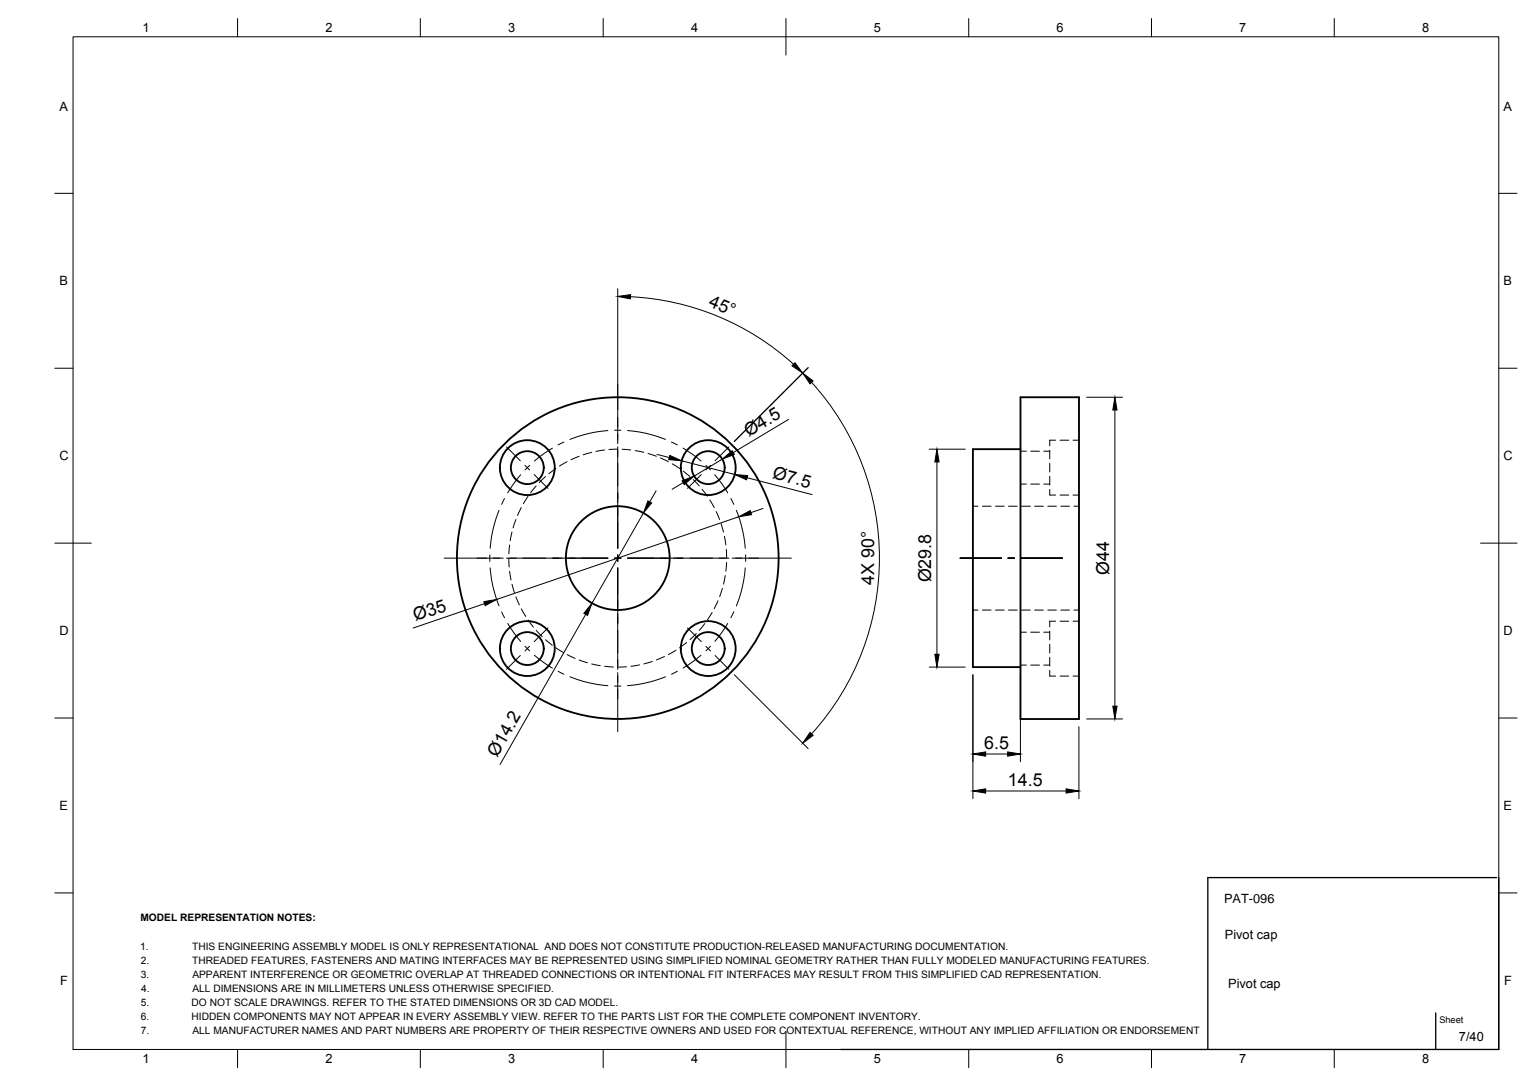
ISO-10303-21;
HEADER;
/* Generated by software containing ST-Developer
 * from STEP Tools, Inc. (www.steptools.com) 
 */

FILE_DESCRIPTION(
/* description */ ('PAT-096'),
/* implementation_level */ '2;1');

FILE_NAME(
/* name */ 'Pivot cap.step',
/* time_stamp */ '2026-10-29T17:03:14-07:00',
/* author */ (''),
/* organization */ (''),
/* preprocessor_version */ 'ST-DEVELOPER v20.2',
/* originating_system */ 'Autodesk Translation Framework v15.17.0.0',
/* authorisation */ '');

FILE_SCHEMA (('AUTOMOTIVE_DESIGN { 1 0 10303 214 3 1 1 }'));
ENDSEC;

DATA;
#10=MECHANICAL_DESIGN_GEOMETRIC_PRESENTATION_REPRESENTATION('',(#401),#10650);
#339=SHAPE_REPRESENTATION_RELATIONSHIP('SRR','None',#10799,#370);
#370=ADVANCED_BREP_SHAPE_REPRESENTATION('',(#439),#10617);
#401=STYLED_ITEM('',(#11050),#439);
#439=MANIFOLD_SOLID_BREP('Body1',#5535);
#508=FACE_BOUND('',#1222,.T.);
#509=FACE_BOUND('',#1225,.T.);
#510=FACE_BOUND('',#1228,.T.);
#511=FACE_BOUND('',#1231,.T.);
#512=FACE_BOUND('',#1238,.T.);
#513=FACE_BOUND('',#1242,.T.);
#514=FACE_BOUND('',#1243,.T.);
#515=FACE_BOUND('',#1244,.T.);
#516=FACE_BOUND('',#1245,.T.);
#517=FACE_BOUND('',#1246,.T.);
#518=FACE_BOUND('',#1248,.T.);
#519=FACE_BOUND('',#1249,.T.);
#520=FACE_BOUND('',#1250,.T.);
#521=FACE_BOUND('',#1251,.T.);
#522=FACE_BOUND('',#1252,.T.);
#641=PLANE('',#6046);
#642=PLANE('',#6051);
#643=PLANE('',#6056);
#644=PLANE('',#6061);
#645=PLANE('',#6074);
#646=PLANE('',#6081);
#647=PLANE('',#6082);
#849=FACE_OUTER_BOUND('',#1220,.T.);
#850=FACE_OUTER_BOUND('',#1221,.T.);
#851=FACE_OUTER_BOUND('',#1223,.T.);
#852=FACE_OUTER_BOUND('',#1224,.T.);
#853=FACE_OUTER_BOUND('',#1226,.T.);
#854=FACE_OUTER_BOUND('',#1227,.T.);
#855=FACE_OUTER_BOUND('',#1229,.T.);
#856=FACE_OUTER_BOUND('',#1230,.T.);
#857=FACE_OUTER_BOUND('',#1232,.T.);
#858=FACE_OUTER_BOUND('',#1233,.T.);
#859=FACE_OUTER_BOUND('',#1234,.T.);
#860=FACE_OUTER_BOUND('',#1235,.T.);
#861=FACE_OUTER_BOUND('',#1236,.T.);
#862=FACE_OUTER_BOUND('',#1237,.T.);
#863=FACE_OUTER_BOUND('',#1239,.T.);
#864=FACE_OUTER_BOUND('',#1240,.T.);
#865=FACE_OUTER_BOUND('',#1241,.T.);
#866=FACE_OUTER_BOUND('',#1247,.T.);
#1220=EDGE_LOOP('',(#3977,#3978,#3979,#3980));
#1221=EDGE_LOOP('',(#3981));
#1222=EDGE_LOOP('',(#3982));
#1223=EDGE_LOOP('',(#3983,#3984,#3985,#3986));
#1224=EDGE_LOOP('',(#3987));
#1225=EDGE_LOOP('',(#3988));
#1226=EDGE_LOOP('',(#3989,#3990,#3991,#3992));
#1227=EDGE_LOOP('',(#3993));
#1228=EDGE_LOOP('',(#3994));
#1229=EDGE_LOOP('',(#3995,#3996,#3997,#3998));
#1230=EDGE_LOOP('',(#3999));
#1231=EDGE_LOOP('',(#4000));
#1232=EDGE_LOOP('',(#4001,#4002,#4003,#4004));
#1233=EDGE_LOOP('',(#4005,#4006,#4007,#4008));
#1234=EDGE_LOOP('',(#4009,#4010,#4011,#4012));
#1235=EDGE_LOOP('',(#4013,#4014,#4015,#4016));
#1236=EDGE_LOOP('',(#4017,#4018,#4019,#4020));
#1237=EDGE_LOOP('',(#4021));
#1238=EDGE_LOOP('',(#4022));
#1239=EDGE_LOOP('',(#4023,#4024,#4025,#4026));
#1240=EDGE_LOOP('',(#4027,#4028,#4029,#4030));
#1241=EDGE_LOOP('',(#4031));
#1242=EDGE_LOOP('',(#4032));
#1243=EDGE_LOOP('',(#4033));
#1244=EDGE_LOOP('',(#4034));
#1245=EDGE_LOOP('',(#4035));
#1246=EDGE_LOOP('',(#4036));
#1247=EDGE_LOOP('',(#4037));
#1248=EDGE_LOOP('',(#4038));
#1249=EDGE_LOOP('',(#4039));
#1250=EDGE_LOOP('',(#4040));
#1251=EDGE_LOOP('',(#4041));
#1252=EDGE_LOOP('',(#4042));
#1665=LINE('',#8867,#1994);
#1666=LINE('',#8876,#1995);
#1667=LINE('',#8885,#1996);
#1668=LINE('',#8894,#1997);
#1669=LINE('',#8902,#1998);
#1670=LINE('',#8906,#1999);
#1671=LINE('',#8910,#2000);
#1672=LINE('',#8914,#2001);
#1673=LINE('',#8919,#2002);
#1674=LINE('',#8927,#2003);
#1675=LINE('',#8932,#2004);
#1994=VECTOR('',#6995,0.375);
#1995=VECTOR('',#7006,0.375);
#1996=VECTOR('',#7017,0.375);
#1997=VECTOR('',#7028,0.375);
#1998=VECTOR('',#7039,0.225);
#1999=VECTOR('',#7044,0.225);
#2000=VECTOR('',#7049,0.225);
#2001=VECTOR('',#7054,0.225);
#2002=VECTOR('',#7059,1.49);
#2003=VECTOR('',#7070,0.71);
#2004=VECTOR('',#7075,2.2);
#2322=CIRCLE('',#6044,0.375);
#2323=CIRCLE('',#6045,0.375);
#2324=CIRCLE('',#6047,0.225);
#2325=CIRCLE('',#6049,0.375);
#2326=CIRCLE('',#6050,0.375);
#2327=CIRCLE('',#6052,0.225);
#2328=CIRCLE('',#6054,0.375);
#2329=CIRCLE('',#6055,0.375);
#2330=CIRCLE('',#6057,0.225);
#2331=CIRCLE('',#6059,0.375);
#2332=CIRCLE('',#6060,0.375);
#2333=CIRCLE('',#6062,0.225);
#2334=CIRCLE('',#6064,0.225);
#2335=CIRCLE('',#6066,0.225);
#2336=CIRCLE('',#6068,0.225);
#2337=CIRCLE('',#6070,0.225);
#2338=CIRCLE('',#6072,1.49);
#2339=CIRCLE('',#6073,1.49);
#2340=CIRCLE('',#6075,0.71);
#2341=CIRCLE('',#6077,0.71);
#2342=CIRCLE('',#6079,2.2);
#2343=CIRCLE('',#6080,2.2);
#2665=VERTEX_POINT('',#8864);
#2666=VERTEX_POINT('',#8866);
#2667=VERTEX_POINT('',#8870);
#2668=VERTEX_POINT('',#8873);
#2669=VERTEX_POINT('',#8875);
#2670=VERTEX_POINT('',#8879);
#2671=VERTEX_POINT('',#8882);
#2672=VERTEX_POINT('',#8884);
#2673=VERTEX_POINT('',#8888);
#2674=VERTEX_POINT('',#8891);
#2675=VERTEX_POINT('',#8893);
#2676=VERTEX_POINT('',#8897);
#2677=VERTEX_POINT('',#8900);
#2678=VERTEX_POINT('',#8904);
#2679=VERTEX_POINT('',#8908);
#2680=VERTEX_POINT('',#8912);
#2681=VERTEX_POINT('',#8916);
#2682=VERTEX_POINT('',#8918);
#2683=VERTEX_POINT('',#8922);
#2684=VERTEX_POINT('',#8925);
#2685=VERTEX_POINT('',#8929);
#2686=VERTEX_POINT('',#8931);
#3167=EDGE_CURVE('',#2665,#2665,#2322,.T.);
#3168=EDGE_CURVE('',#2665,#2666,#1665,.T.);
#3169=EDGE_CURVE('',#2666,#2666,#2323,.T.);
#3170=EDGE_CURVE('',#2667,#2667,#2324,.T.);
#3171=EDGE_CURVE('',#2668,#2668,#2325,.T.);
#3172=EDGE_CURVE('',#2668,#2669,#1666,.T.);
#3173=EDGE_CURVE('',#2669,#2669,#2326,.T.);
#3174=EDGE_CURVE('',#2670,#2670,#2327,.T.);
#3175=EDGE_CURVE('',#2671,#2671,#2328,.T.);
#3176=EDGE_CURVE('',#2671,#2672,#1667,.T.);
#3177=EDGE_CURVE('',#2672,#2672,#2329,.T.);
#3178=EDGE_CURVE('',#2673,#2673,#2330,.T.);
#3179=EDGE_CURVE('',#2674,#2674,#2331,.T.);
#3180=EDGE_CURVE('',#2674,#2675,#1668,.T.);
#3181=EDGE_CURVE('',#2675,#2675,#2332,.T.);
#3182=EDGE_CURVE('',#2676,#2676,#2333,.T.);
#3183=EDGE_CURVE('',#2677,#2677,#2334,.T.);
#3184=EDGE_CURVE('',#2677,#2667,#1669,.T.);
#3185=EDGE_CURVE('',#2678,#2678,#2335,.T.);
#3186=EDGE_CURVE('',#2678,#2670,#1670,.T.);
#3187=EDGE_CURVE('',#2679,#2679,#2336,.T.);
#3188=EDGE_CURVE('',#2679,#2673,#1671,.T.);
#3189=EDGE_CURVE('',#2680,#2680,#2337,.T.);
#3190=EDGE_CURVE('',#2680,#2676,#1672,.T.);
#3191=EDGE_CURVE('',#2681,#2681,#2338,.T.);
#3192=EDGE_CURVE('',#2681,#2682,#1673,.T.);
#3193=EDGE_CURVE('',#2682,#2682,#2339,.T.);
#3194=EDGE_CURVE('',#2683,#2683,#2340,.T.);
#3195=EDGE_CURVE('',#2684,#2684,#2341,.T.);
#3196=EDGE_CURVE('',#2684,#2683,#1674,.T.);
#3197=EDGE_CURVE('',#2685,#2685,#2342,.T.);
#3198=EDGE_CURVE('',#2685,#2686,#1675,.T.);
#3199=EDGE_CURVE('',#2686,#2686,#2343,.T.);
#3977=ORIENTED_EDGE('',*,*,#3167,.F.);
#3978=ORIENTED_EDGE('',*,*,#3168,.T.);
#3979=ORIENTED_EDGE('',*,*,#3169,.F.);
#3980=ORIENTED_EDGE('',*,*,#3168,.F.);
#3981=ORIENTED_EDGE('',*,*,#3167,.T.);
#3982=ORIENTED_EDGE('',*,*,#3170,.F.);
#3983=ORIENTED_EDGE('',*,*,#3171,.F.);
#3984=ORIENTED_EDGE('',*,*,#3172,.T.);
#3985=ORIENTED_EDGE('',*,*,#3173,.F.);
#3986=ORIENTED_EDGE('',*,*,#3172,.F.);
#3987=ORIENTED_EDGE('',*,*,#3171,.T.);
#3988=ORIENTED_EDGE('',*,*,#3174,.F.);
#3989=ORIENTED_EDGE('',*,*,#3175,.F.);
#3990=ORIENTED_EDGE('',*,*,#3176,.T.);
#3991=ORIENTED_EDGE('',*,*,#3177,.F.);
#3992=ORIENTED_EDGE('',*,*,#3176,.F.);
#3993=ORIENTED_EDGE('',*,*,#3175,.T.);
#3994=ORIENTED_EDGE('',*,*,#3178,.F.);
#3995=ORIENTED_EDGE('',*,*,#3179,.F.);
#3996=ORIENTED_EDGE('',*,*,#3180,.T.);
#3997=ORIENTED_EDGE('',*,*,#3181,.F.);
#3998=ORIENTED_EDGE('',*,*,#3180,.F.);
#3999=ORIENTED_EDGE('',*,*,#3179,.T.);
#4000=ORIENTED_EDGE('',*,*,#3182,.F.);
#4001=ORIENTED_EDGE('',*,*,#3183,.F.);
#4002=ORIENTED_EDGE('',*,*,#3184,.T.);
#4003=ORIENTED_EDGE('',*,*,#3170,.T.);
#4004=ORIENTED_EDGE('',*,*,#3184,.F.);
#4005=ORIENTED_EDGE('',*,*,#3185,.F.);
#4006=ORIENTED_EDGE('',*,*,#3186,.T.);
#4007=ORIENTED_EDGE('',*,*,#3174,.T.);
#4008=ORIENTED_EDGE('',*,*,#3186,.F.);
#4009=ORIENTED_EDGE('',*,*,#3187,.F.);
#4010=ORIENTED_EDGE('',*,*,#3188,.T.);
#4011=ORIENTED_EDGE('',*,*,#3178,.T.);
#4012=ORIENTED_EDGE('',*,*,#3188,.F.);
#4013=ORIENTED_EDGE('',*,*,#3189,.F.);
#4014=ORIENTED_EDGE('',*,*,#3190,.T.);
#4015=ORIENTED_EDGE('',*,*,#3182,.T.);
#4016=ORIENTED_EDGE('',*,*,#3190,.F.);
#4017=ORIENTED_EDGE('',*,*,#3191,.F.);
#4018=ORIENTED_EDGE('',*,*,#3192,.T.);
#4019=ORIENTED_EDGE('',*,*,#3193,.T.);
#4020=ORIENTED_EDGE('',*,*,#3192,.F.);
#4021=ORIENTED_EDGE('',*,*,#3193,.F.);
#4022=ORIENTED_EDGE('',*,*,#3194,.F.);
#4023=ORIENTED_EDGE('',*,*,#3195,.F.);
#4024=ORIENTED_EDGE('',*,*,#3196,.T.);
#4025=ORIENTED_EDGE('',*,*,#3194,.T.);
#4026=ORIENTED_EDGE('',*,*,#3196,.F.);
#4027=ORIENTED_EDGE('',*,*,#3197,.F.);
#4028=ORIENTED_EDGE('',*,*,#3198,.T.);
#4029=ORIENTED_EDGE('',*,*,#3199,.T.);
#4030=ORIENTED_EDGE('',*,*,#3198,.F.);
#4031=ORIENTED_EDGE('',*,*,#3197,.T.);
#4032=ORIENTED_EDGE('',*,*,#3195,.T.);
#4033=ORIENTED_EDGE('',*,*,#3181,.T.);
#4034=ORIENTED_EDGE('',*,*,#3177,.T.);
#4035=ORIENTED_EDGE('',*,*,#3173,.T.);
#4036=ORIENTED_EDGE('',*,*,#3169,.T.);
#4037=ORIENTED_EDGE('',*,*,#3199,.F.);
#4038=ORIENTED_EDGE('',*,*,#3191,.T.);
#4039=ORIENTED_EDGE('',*,*,#3189,.T.);
#4040=ORIENTED_EDGE('',*,*,#3187,.T.);
#4041=ORIENTED_EDGE('',*,*,#3185,.T.);
#4042=ORIENTED_EDGE('',*,*,#3183,.T.);
#5100=CYLINDRICAL_SURFACE('',#6043,0.375);
#5101=CYLINDRICAL_SURFACE('',#6048,0.375);
#5102=CYLINDRICAL_SURFACE('',#6053,0.375);
#5103=CYLINDRICAL_SURFACE('',#6058,0.375);
#5104=CYLINDRICAL_SURFACE('',#6063,0.225);
#5105=CYLINDRICAL_SURFACE('',#6065,0.225);
#5106=CYLINDRICAL_SURFACE('',#6067,0.225);
#5107=CYLINDRICAL_SURFACE('',#6069,0.225);
#5108=CYLINDRICAL_SURFACE('',#6071,1.49);
#5109=CYLINDRICAL_SURFACE('',#6076,0.71);
#5110=CYLINDRICAL_SURFACE('',#6078,2.2);
#5254=ADVANCED_FACE('',(#849),#5100,.F.);
#5255=ADVANCED_FACE('',(#850,#508),#641,.T.);
#5256=ADVANCED_FACE('',(#851),#5101,.F.);
#5257=ADVANCED_FACE('',(#852,#509),#642,.T.);
#5258=ADVANCED_FACE('',(#853),#5102,.F.);
#5259=ADVANCED_FACE('',(#854,#510),#643,.T.);
#5260=ADVANCED_FACE('',(#855),#5103,.F.);
#5261=ADVANCED_FACE('',(#856,#511),#644,.T.);
#5262=ADVANCED_FACE('',(#857),#5104,.F.);
#5263=ADVANCED_FACE('',(#858),#5105,.F.);
#5264=ADVANCED_FACE('',(#859),#5106,.F.);
#5265=ADVANCED_FACE('',(#860),#5107,.F.);
#5266=ADVANCED_FACE('',(#861),#5108,.T.);
#5267=ADVANCED_FACE('',(#862,#512),#645,.F.);
#5268=ADVANCED_FACE('',(#863),#5109,.F.);
#5269=ADVANCED_FACE('',(#864),#5110,.T.);
#5270=ADVANCED_FACE('',(#865,#513,#514,#515,#516,#517),#646,.T.);
#5271=ADVANCED_FACE('',(#866,#518,#519,#520,#521,#522),#647,.F.);
#5535=CLOSED_SHELL('',(#5254,#5255,#5256,#5257,#5258,#5259,#5260,#5261,
#5262,#5263,#5264,#5265,#5266,#5267,#5268,#5269,#5270,#5271));
#6042=AXIS2_PLACEMENT_3D('',#8862,#6989,#6990);
#6043=AXIS2_PLACEMENT_3D('',#8863,#6991,#6992);
#6044=AXIS2_PLACEMENT_3D('',#8865,#6993,#6994);
#6045=AXIS2_PLACEMENT_3D('',#8868,#6996,#6997);
#6046=AXIS2_PLACEMENT_3D('',#8869,#6998,#6999);
#6047=AXIS2_PLACEMENT_3D('',#8871,#7000,#7001);
#6048=AXIS2_PLACEMENT_3D('',#8872,#7002,#7003);
#6049=AXIS2_PLACEMENT_3D('',#8874,#7004,#7005);
#6050=AXIS2_PLACEMENT_3D('',#8877,#7007,#7008);
#6051=AXIS2_PLACEMENT_3D('',#8878,#7009,#7010);
#6052=AXIS2_PLACEMENT_3D('',#8880,#7011,#7012);
#6053=AXIS2_PLACEMENT_3D('',#8881,#7013,#7014);
#6054=AXIS2_PLACEMENT_3D('',#8883,#7015,#7016);
#6055=AXIS2_PLACEMENT_3D('',#8886,#7018,#7019);
#6056=AXIS2_PLACEMENT_3D('',#8887,#7020,#7021);
#6057=AXIS2_PLACEMENT_3D('',#8889,#7022,#7023);
#6058=AXIS2_PLACEMENT_3D('',#8890,#7024,#7025);
#6059=AXIS2_PLACEMENT_3D('',#8892,#7026,#7027);
#6060=AXIS2_PLACEMENT_3D('',#8895,#7029,#7030);
#6061=AXIS2_PLACEMENT_3D('',#8896,#7031,#7032);
#6062=AXIS2_PLACEMENT_3D('',#8898,#7033,#7034);
#6063=AXIS2_PLACEMENT_3D('',#8899,#7035,#7036);
#6064=AXIS2_PLACEMENT_3D('',#8901,#7037,#7038);
#6065=AXIS2_PLACEMENT_3D('',#8903,#7040,#7041);
#6066=AXIS2_PLACEMENT_3D('',#8905,#7042,#7043);
#6067=AXIS2_PLACEMENT_3D('',#8907,#7045,#7046);
#6068=AXIS2_PLACEMENT_3D('',#8909,#7047,#7048);
#6069=AXIS2_PLACEMENT_3D('',#8911,#7050,#7051);
#6070=AXIS2_PLACEMENT_3D('',#8913,#7052,#7053);
#6071=AXIS2_PLACEMENT_3D('',#8915,#7055,#7056);
#6072=AXIS2_PLACEMENT_3D('',#8917,#7057,#7058);
#6073=AXIS2_PLACEMENT_3D('',#8920,#7060,#7061);
#6074=AXIS2_PLACEMENT_3D('',#8921,#7062,#7063);
#6075=AXIS2_PLACEMENT_3D('',#8923,#7064,#7065);
#6076=AXIS2_PLACEMENT_3D('',#8924,#7066,#7067);
#6077=AXIS2_PLACEMENT_3D('',#8926,#7068,#7069);
#6078=AXIS2_PLACEMENT_3D('',#8928,#7071,#7072);
#6079=AXIS2_PLACEMENT_3D('',#8930,#7073,#7074);
#6080=AXIS2_PLACEMENT_3D('',#8933,#7076,#7077);
#6081=AXIS2_PLACEMENT_3D('',#8934,#7078,#7079);
#6082=AXIS2_PLACEMENT_3D('',#8935,#7080,#7081);
#6989=DIRECTION('axis',(0.,0.,1.));
#6990=DIRECTION('refdir',(1.,0.,0.));
#6991=DIRECTION('center_axis',(0.,0.,1.));
#6992=DIRECTION('ref_axis',(1.,0.,0.));
#6993=DIRECTION('center_axis',(0.,0.,1.));
#6994=DIRECTION('ref_axis',(1.,0.,0.));
#6995=DIRECTION('',(0.,0.,1.));
#6996=DIRECTION('center_axis',(0.,0.,-1.));
#6997=DIRECTION('ref_axis',(1.,0.,0.));
#6998=DIRECTION('center_axis',(0.,0.,1.));
#6999=DIRECTION('ref_axis',(1.,0.,0.));
#7000=DIRECTION('center_axis',(0.,0.,1.));
#7001=DIRECTION('ref_axis',(1.,0.,0.));
#7002=DIRECTION('center_axis',(0.,0.,1.));
#7003=DIRECTION('ref_axis',(1.,0.,0.));
#7004=DIRECTION('center_axis',(0.,0.,1.));
#7005=DIRECTION('ref_axis',(1.,0.,0.));
#7006=DIRECTION('',(0.,0.,1.));
#7007=DIRECTION('center_axis',(0.,0.,-1.));
#7008=DIRECTION('ref_axis',(1.,0.,0.));
#7009=DIRECTION('center_axis',(0.,0.,1.));
#7010=DIRECTION('ref_axis',(1.,0.,0.));
#7011=DIRECTION('center_axis',(0.,0.,1.));
#7012=DIRECTION('ref_axis',(1.,0.,0.));
#7013=DIRECTION('center_axis',(0.,0.,1.));
#7014=DIRECTION('ref_axis',(1.,0.,0.));
#7015=DIRECTION('center_axis',(0.,0.,1.));
#7016=DIRECTION('ref_axis',(1.,0.,0.));
#7017=DIRECTION('',(0.,0.,1.));
#7018=DIRECTION('center_axis',(0.,0.,-1.));
#7019=DIRECTION('ref_axis',(1.,0.,0.));
#7020=DIRECTION('center_axis',(0.,0.,1.));
#7021=DIRECTION('ref_axis',(1.,0.,0.));
#7022=DIRECTION('center_axis',(0.,0.,1.));
#7023=DIRECTION('ref_axis',(1.,0.,0.));
#7024=DIRECTION('center_axis',(0.,0.,1.));
#7025=DIRECTION('ref_axis',(1.,0.,0.));
#7026=DIRECTION('center_axis',(0.,0.,1.));
#7027=DIRECTION('ref_axis',(1.,0.,0.));
#7028=DIRECTION('',(0.,0.,1.));
#7029=DIRECTION('center_axis',(0.,0.,-1.));
#7030=DIRECTION('ref_axis',(1.,0.,0.));
#7031=DIRECTION('center_axis',(0.,0.,1.));
#7032=DIRECTION('ref_axis',(1.,0.,0.));
#7033=DIRECTION('center_axis',(0.,0.,1.));
#7034=DIRECTION('ref_axis',(1.,0.,0.));
#7035=DIRECTION('center_axis',(0.,0.,1.));
#7036=DIRECTION('ref_axis',(1.,0.,0.));
#7037=DIRECTION('center_axis',(0.,0.,1.));
#7038=DIRECTION('ref_axis',(1.,0.,0.));
#7039=DIRECTION('',(0.,0.,1.));
#7040=DIRECTION('center_axis',(0.,0.,1.));
#7041=DIRECTION('ref_axis',(1.,0.,0.));
#7042=DIRECTION('center_axis',(0.,0.,1.));
#7043=DIRECTION('ref_axis',(1.,0.,0.));
#7044=DIRECTION('',(0.,0.,1.));
#7045=DIRECTION('center_axis',(0.,0.,1.));
#7046=DIRECTION('ref_axis',(1.,0.,0.));
#7047=DIRECTION('center_axis',(0.,0.,1.));
#7048=DIRECTION('ref_axis',(1.,0.,0.));
#7049=DIRECTION('',(0.,0.,1.));
#7050=DIRECTION('center_axis',(0.,0.,1.));
#7051=DIRECTION('ref_axis',(1.,0.,0.));
#7052=DIRECTION('center_axis',(0.,0.,1.));
#7053=DIRECTION('ref_axis',(1.,0.,0.));
#7054=DIRECTION('',(0.,0.,1.));
#7055=DIRECTION('center_axis',(0.,0.,1.));
#7056=DIRECTION('ref_axis',(1.,0.,0.));
#7057=DIRECTION('center_axis',(0.,0.,1.));
#7058=DIRECTION('ref_axis',(1.,0.,0.));
#7059=DIRECTION('',(0.,0.,-1.));
#7060=DIRECTION('center_axis',(0.,0.,1.));
#7061=DIRECTION('ref_axis',(1.,0.,0.));
#7062=DIRECTION('center_axis',(0.,0.,1.));
#7063=DIRECTION('ref_axis',(1.,0.,0.));
#7064=DIRECTION('center_axis',(0.,0.,-1.));
#7065=DIRECTION('ref_axis',(1.,0.,0.));
#7066=DIRECTION('center_axis',(0.,0.,1.));
#7067=DIRECTION('ref_axis',(1.,0.,0.));
#7068=DIRECTION('center_axis',(0.,0.,-1.));
#7069=DIRECTION('ref_axis',(1.,0.,0.));
#7070=DIRECTION('',(0.,0.,-1.));
#7071=DIRECTION('center_axis',(0.,0.,1.));
#7072=DIRECTION('ref_axis',(1.,0.,0.));
#7073=DIRECTION('center_axis',(0.,0.,1.));
#7074=DIRECTION('ref_axis',(1.,0.,0.));
#7075=DIRECTION('',(0.,0.,-1.));
#7076=DIRECTION('center_axis',(0.,0.,1.));
#7077=DIRECTION('ref_axis',(1.,0.,0.));
#7078=DIRECTION('center_axis',(0.,0.,1.));
#7079=DIRECTION('ref_axis',(1.,0.,0.));
#7080=DIRECTION('center_axis',(0.,0.,1.));
#7081=DIRECTION('ref_axis',(1.,0.,0.));
#8862=CARTESIAN_POINT('',(0.,0.,0.));
#8863=CARTESIAN_POINT('Origin',(-1.23743686707646,-1.23743686707646,4.));
#8864=CARTESIAN_POINT('',(-1.61243686707646,-1.23743686707646,4.));
#8865=CARTESIAN_POINT('Origin',(-1.23743686707646,-1.23743686707646,4.));
#8866=CARTESIAN_POINT('',(-1.61243686707646,-1.23743686707646,4.4));
#8867=CARTESIAN_POINT('',(-1.61243686707646,-1.23743686707646,4.));
#8868=CARTESIAN_POINT('Origin',(-1.23743686707646,-1.23743686707646,4.4));
#8869=CARTESIAN_POINT('Origin',(-1.23743686707646,-1.23743686707646,4.));
#8870=CARTESIAN_POINT('',(-1.46243686707646,-1.23743686707646,4.));
#8871=CARTESIAN_POINT('Origin',(-1.23743686707646,-1.23743686707646,4.));
#8872=CARTESIAN_POINT('Origin',(-1.23743686707646,1.23743686707646,4.));
#8873=CARTESIAN_POINT('',(-1.61243686707646,1.23743686707646,4.));
#8874=CARTESIAN_POINT('Origin',(-1.23743686707646,1.23743686707646,4.));
#8875=CARTESIAN_POINT('',(-1.61243686707646,1.23743686707646,4.4));
#8876=CARTESIAN_POINT('',(-1.61243686707646,1.23743686707646,4.));
#8877=CARTESIAN_POINT('Origin',(-1.23743686707646,1.23743686707646,4.4));
#8878=CARTESIAN_POINT('Origin',(-1.23743686707646,1.23743686707646,4.));
#8879=CARTESIAN_POINT('',(-1.46243686707646,1.23743686707646,4.));
#8880=CARTESIAN_POINT('Origin',(-1.23743686707646,1.23743686707646,4.));
#8881=CARTESIAN_POINT('Origin',(1.23743686707646,1.23743686707646,4.));
#8882=CARTESIAN_POINT('',(0.862436867076458,1.23743686707646,4.));
#8883=CARTESIAN_POINT('Origin',(1.23743686707646,1.23743686707646,4.));
#8884=CARTESIAN_POINT('',(0.862436867076458,1.23743686707646,4.4));
#8885=CARTESIAN_POINT('',(0.862436867076458,1.23743686707646,4.));
#8886=CARTESIAN_POINT('Origin',(1.23743686707646,1.23743686707646,4.4));
#8887=CARTESIAN_POINT('Origin',(1.23743686707646,1.23743686707646,4.));
#8888=CARTESIAN_POINT('',(1.01243686707646,1.23743686707646,4.));
#8889=CARTESIAN_POINT('Origin',(1.23743686707646,1.23743686707646,4.));
#8890=CARTESIAN_POINT('Origin',(1.23743686707646,-1.23743686707646,4.));
#8891=CARTESIAN_POINT('',(0.862436867076458,-1.23743686707646,4.));
#8892=CARTESIAN_POINT('Origin',(1.23743686707646,-1.23743686707646,4.));
#8893=CARTESIAN_POINT('',(0.862436867076458,-1.23743686707646,4.4));
#8894=CARTESIAN_POINT('',(0.862436867076458,-1.23743686707646,4.));
#8895=CARTESIAN_POINT('Origin',(1.23743686707646,-1.23743686707646,4.4));
#8896=CARTESIAN_POINT('Origin',(1.23743686707646,-1.23743686707646,4.));
#8897=CARTESIAN_POINT('',(1.01243686707646,-1.23743686707646,4.));
#8898=CARTESIAN_POINT('Origin',(1.23743686707646,-1.23743686707646,4.));
#8899=CARTESIAN_POINT('Origin',(-1.23743686707646,-1.23743686707646,3.5));
#8900=CARTESIAN_POINT('',(-1.46243686707646,-1.23743686707646,3.6));
#8901=CARTESIAN_POINT('Origin',(-1.23743686707646,-1.23743686707646,3.6));
#8902=CARTESIAN_POINT('',(-1.46243686707646,-1.23743686707646,3.5));
#8903=CARTESIAN_POINT('Origin',(-1.23743686707646,1.23743686707646,3.5));
#8904=CARTESIAN_POINT('',(-1.46243686707646,1.23743686707646,3.6));
#8905=CARTESIAN_POINT('Origin',(-1.23743686707646,1.23743686707646,3.6));
#8906=CARTESIAN_POINT('',(-1.46243686707646,1.23743686707646,3.5));
#8907=CARTESIAN_POINT('Origin',(1.23743686707646,1.23743686707646,3.5));
#8908=CARTESIAN_POINT('',(1.01243686707646,1.23743686707646,3.6));
#8909=CARTESIAN_POINT('Origin',(1.23743686707646,1.23743686707646,3.6));
#8910=CARTESIAN_POINT('',(1.01243686707646,1.23743686707646,3.5));
#8911=CARTESIAN_POINT('Origin',(1.23743686707646,-1.23743686707646,3.5));
#8912=CARTESIAN_POINT('',(1.01243686707646,-1.23743686707646,3.6));
#8913=CARTESIAN_POINT('Origin',(1.23743686707646,-1.23743686707646,3.6));
#8914=CARTESIAN_POINT('',(1.01243686707646,-1.23743686707646,3.5));
#8915=CARTESIAN_POINT('Origin',(0.,0.,2.95));
#8916=CARTESIAN_POINT('',(-1.49,-1.82472373072956E-16,3.6));
#8917=CARTESIAN_POINT('Origin',(0.,0.,3.6));
#8918=CARTESIAN_POINT('',(-1.49,-1.82472373072956E-16,2.95));
#8919=CARTESIAN_POINT('',(-1.49,-1.82472373072956E-16,2.95));
#8920=CARTESIAN_POINT('Origin',(0.,0.,2.95));
#8921=CARTESIAN_POINT('Origin',(0.,0.,2.95));
#8922=CARTESIAN_POINT('',(-0.71,-8.69499227394621E-17,2.95));
#8923=CARTESIAN_POINT('Origin',(0.,0.,2.95));
#8924=CARTESIAN_POINT('Origin',(0.,0.,3.6));
#8925=CARTESIAN_POINT('',(-0.71,-8.69499227394621E-17,4.4));
#8926=CARTESIAN_POINT('Origin',(0.,0.,4.4));
#8927=CARTESIAN_POINT('',(-0.71,-8.69499227394621E-17,3.6));
#8928=CARTESIAN_POINT('Origin',(0.,0.,3.6));
#8929=CARTESIAN_POINT('',(-2.2,-2.69422295812418E-16,4.4));
#8930=CARTESIAN_POINT('Origin',(0.,0.,4.4));
#8931=CARTESIAN_POINT('',(-2.2,-2.69422295812418E-16,3.6));
#8932=CARTESIAN_POINT('',(-2.2,-2.69422295812418E-16,3.6));
#8933=CARTESIAN_POINT('Origin',(0.,0.,3.6));
#8934=CARTESIAN_POINT('Origin',(0.,0.,4.4));
#8935=CARTESIAN_POINT('Origin',(0.,0.,3.6));
#10578=UNCERTAINTY_MEASURE_WITH_UNIT(LENGTH_MEASURE(0.001),#10651,
'DISTANCE_ACCURACY_VALUE',
'Maximum model space distance between geometric entities at asserted c
onnectivities');
#10611=UNCERTAINTY_MEASURE_WITH_UNIT(LENGTH_MEASURE(0.001),#10651,
'DISTANCE_ACCURACY_VALUE',
'Maximum model space distance between geometric entities at asserted c
onnectivities');
#10617=(
GEOMETRIC_REPRESENTATION_CONTEXT(3)
GLOBAL_UNCERTAINTY_ASSIGNED_CONTEXT((#10578))
GLOBAL_UNIT_ASSIGNED_CONTEXT((#10651,#10653,#10654))
REPRESENTATION_CONTEXT('','3D')
);
#10650=(
GEOMETRIC_REPRESENTATION_CONTEXT(3)
GLOBAL_UNCERTAINTY_ASSIGNED_CONTEXT((#10611))
GLOBAL_UNIT_ASSIGNED_CONTEXT((#10651,#10653,#10654))
REPRESENTATION_CONTEXT('','3D')
);
#10651=(
LENGTH_UNIT()
NAMED_UNIT(*)
SI_UNIT(.CENTI.,.METRE.)
);
#10653=(
NAMED_UNIT(*)
PLANE_ANGLE_UNIT()
SI_UNIT($,.RADIAN.)
);
#10654=(
NAMED_UNIT(*)
SI_UNIT($,.STERADIAN.)
SOLID_ANGLE_UNIT()
);
#10660=SHAPE_DEFINITION_REPRESENTATION(#10698,#10799);
#10698=PRODUCT_DEFINITION_SHAPE('',$,#10838);
#10799=SHAPE_REPRESENTATION('',(#6042),#10617);
#10832=PRODUCT_DEFINITION_CONTEXT('part definition',#10948,'design');
#10838=PRODUCT_DEFINITION('Pivot cap','Pivot cap',#10876,#10832);
#10876=PRODUCT_DEFINITION_FORMATION('',$,#10955);
#10948=APPLICATION_CONTEXT(
'Core Data for Automotive Mechanical Design Process');
#10949=PRODUCT_CONTEXT('part definition',#10948,'mechanical');
#10955=PRODUCT('Pivot cap','Pivot cap','Pivot cap',(#10949));
#11044=COLOUR_RGB('Light Blue',0.38,0.62,0.78);
#11045=FILL_AREA_STYLE_COLOUR('',#11044);
#11046=FILL_AREA_STYLE('',(#11045));
#11047=SURFACE_STYLE_FILL_AREA(#11046);
#11048=SURFACE_SIDE_STYLE('',(#11047));
#11049=SURFACE_STYLE_USAGE(.BOTH.,#11048);
#11050=PRESENTATION_STYLE_ASSIGNMENT((#11049));
ENDSEC;
END-ISO-10303-21;
